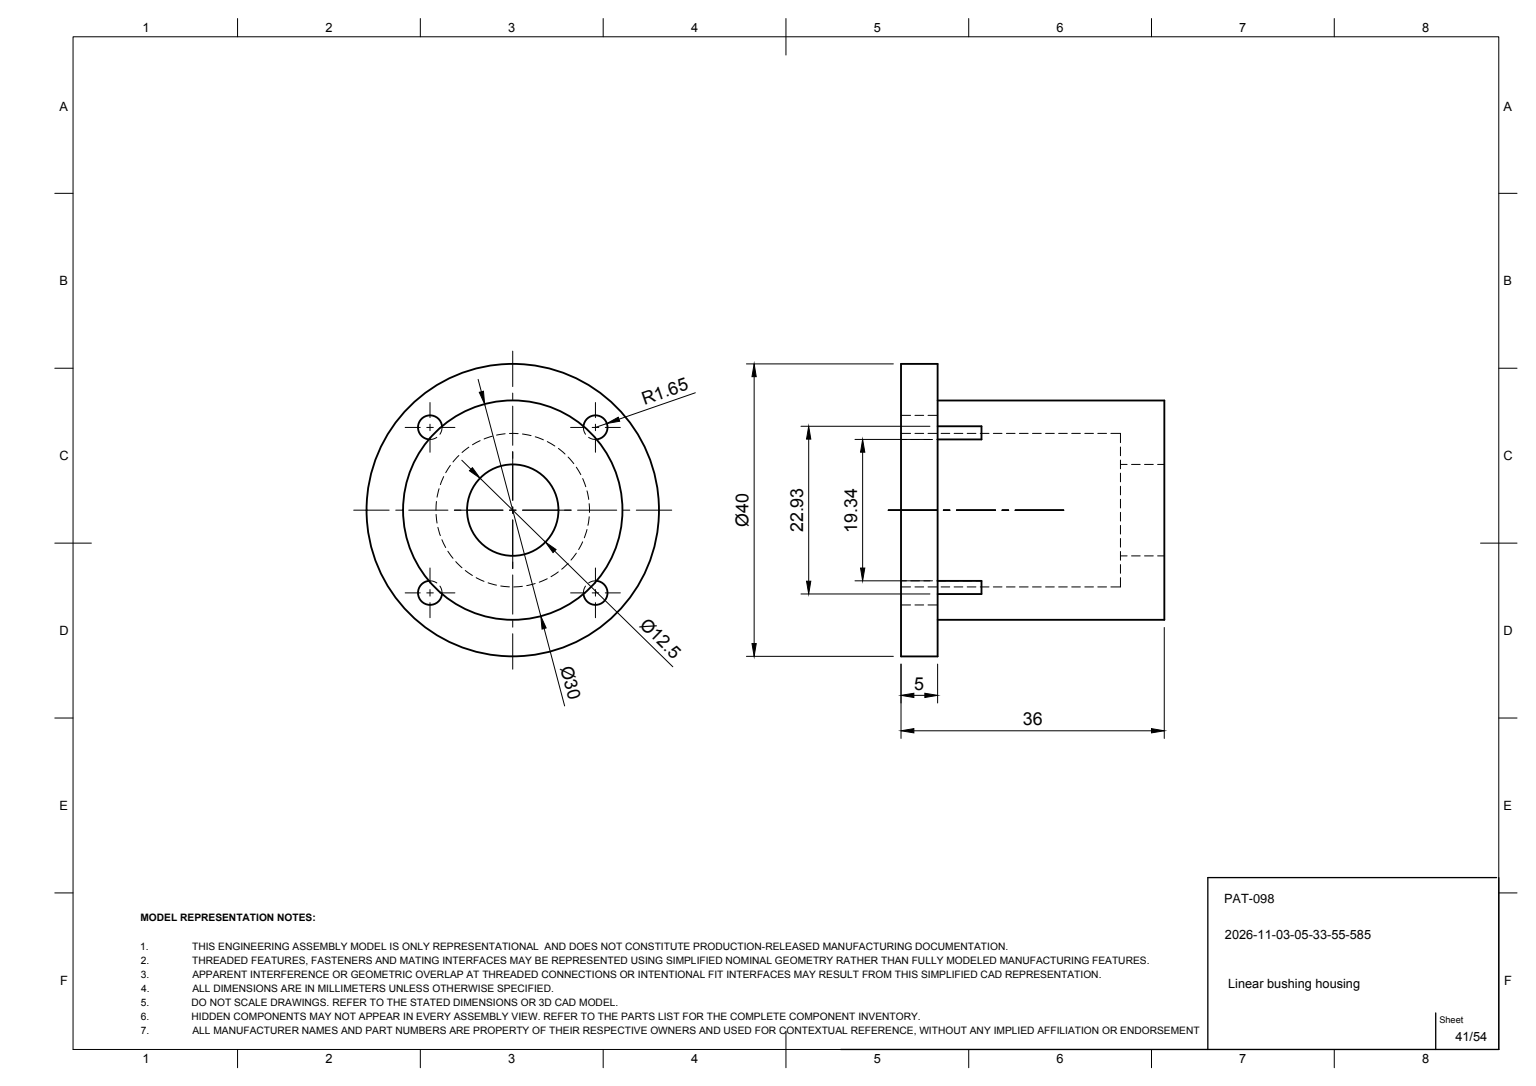
ISO-10303-21;
HEADER;
/* Generated by software containing ST-Developer
 * from STEP Tools, Inc. (www.steptools.com) 
 */

FILE_DESCRIPTION(
/* description */ ('Spring compression tester'),
/* implementation_level */ '2;1');

FILE_NAME(
/* name */ 'Linear bushing housing.step',
/* time_stamp */ '2026-10-28T03:24:11-07:00',
/* author */ (''),
/* organization */ (''),
/* preprocessor_version */ 'ST-DEVELOPER v20.2',
/* originating_system */ 'Autodesk Translation Framework v15.17.0.0',
/* authorisation */ '');

FILE_SCHEMA (('AUTOMOTIVE_DESIGN { 1 0 10303 214 3 1 1 }'));
ENDSEC;

DATA;
#10=MECHANICAL_DESIGN_GEOMETRIC_PRESENTATION_REPRESENTATION('',(#1159),#43521);
#1024=SHAPE_REPRESENTATION_RELATIONSHIP('SRR','None',#43839,#1084);
#1084=ADVANCED_BREP_SHAPE_REPRESENTATION('',(#1230),#43499);
#1159=STYLED_ITEM('',(#44181),#1230);
#1230=MANIFOLD_SOLID_BREP('Body1',#18600);
#1513=FACE_BOUND('',#4170,.T.);
#1514=FACE_BOUND('',#4172,.T.);
#1515=FACE_BOUND('',#4176,.T.);
#1516=FACE_BOUND('',#4177,.T.);
#1517=FACE_BOUND('',#4178,.T.);
#1518=FACE_BOUND('',#4179,.T.);
#1519=FACE_BOUND('',#4180,.T.);
#1520=FACE_BOUND('',#4182,.T.);
#2030=PLANE('',#20489);
#2031=PLANE('',#20496);
#2032=PLANE('',#20503);
#2033=PLANE('',#20510);
#2034=PLANE('',#20527);
#2035=PLANE('',#20529);
#2036=PLANE('',#20535);
#2037=PLANE('',#20536);
#2846=FACE_OUTER_BOUND('',#4159,.T.);
#2847=FACE_OUTER_BOUND('',#4160,.T.);
#2848=FACE_OUTER_BOUND('',#4161,.T.);
#2849=FACE_OUTER_BOUND('',#4162,.T.);
#2850=FACE_OUTER_BOUND('',#4163,.T.);
#2851=FACE_OUTER_BOUND('',#4164,.T.);
#2852=FACE_OUTER_BOUND('',#4165,.T.);
#2853=FACE_OUTER_BOUND('',#4166,.T.);
#2854=FACE_OUTER_BOUND('',#4167,.T.);
#2855=FACE_OUTER_BOUND('',#4168,.T.);
#2856=FACE_OUTER_BOUND('',#4169,.T.);
#2857=FACE_OUTER_BOUND('',#4171,.T.);
#2858=FACE_OUTER_BOUND('',#4173,.T.);
#2859=FACE_OUTER_BOUND('',#4174,.T.);
#2860=FACE_OUTER_BOUND('',#4175,.T.);
#2861=FACE_OUTER_BOUND('',#4181,.T.);
#4159=EDGE_LOOP('',(#15261,#15262));
#4160=EDGE_LOOP('',(#15263,#15264,#15265,#15266,#15267,#15268,#15269,#15270));
#4161=EDGE_LOOP('',(#15271,#15272));
#4162=EDGE_LOOP('',(#15273,#15274,#15275,#15276,#15277,#15278,#15279,#15280));
#4163=EDGE_LOOP('',(#15281,#15282,#15283));
#4164=EDGE_LOOP('',(#15284,#15285,#15286,#15287,#15288,#15289,#15290,#15291));
#4165=EDGE_LOOP('',(#15292,#15293,#15294));
#4166=EDGE_LOOP('',(#15295,#15296,#15297,#15298,#15299,#15300,#15301,#15302));
#4167=EDGE_LOOP('',(#15303,#15304,#15305,#15306,#15307,#15308,#15309,#15310,
#15311,#15312,#15313,#15314,#15315,#15316,#15317,#15318,#15319,#15320,#15321,
#15322));
#4168=EDGE_LOOP('',(#15323,#15324,#15325,#15326));
#4169=EDGE_LOOP('',(#15327));
#4170=EDGE_LOOP('',(#15328));
#4171=EDGE_LOOP('',(#15329));
#4172=EDGE_LOOP('',(#15330,#15331,#15332,#15333,#15334,#15335,#15336,#15337,
#15338,#15339,#15340));
#4173=EDGE_LOOP('',(#15341,#15342,#15343,#15344));
#4174=EDGE_LOOP('',(#15345,#15346,#15347,#15348));
#4175=EDGE_LOOP('',(#15349));
#4176=EDGE_LOOP('',(#15350));
#4177=EDGE_LOOP('',(#15351));
#4178=EDGE_LOOP('',(#15352));
#4179=EDGE_LOOP('',(#15353));
#4180=EDGE_LOOP('',(#15354));
#4181=EDGE_LOOP('',(#15355));
#4182=EDGE_LOOP('',(#15356));
#5623=LINE('',#30371,#7055);
#5624=LINE('',#30375,#7056);
#5625=LINE('',#30379,#7057);
#5626=LINE('',#30387,#7058);
#5627=LINE('',#30391,#7059);
#5628=LINE('',#30395,#7060);
#5629=LINE('',#30405,#7061);
#5630=LINE('',#30408,#7062);
#5631=LINE('',#30410,#7063);
#5632=LINE('',#30421,#7064);
#5633=LINE('',#30424,#7065);
#5634=LINE('',#30426,#7066);
#5635=LINE('',#30432,#7067);
#5636=LINE('',#30442,#7068);
#5637=LINE('',#30453,#7069);
#5638=LINE('',#30456,#7070);
#7055=VECTOR('',#24631,1.);
#7056=VECTOR('',#24634,0.165);
#7057=VECTOR('',#24639,1.);
#7058=VECTOR('',#24648,1.);
#7059=VECTOR('',#24651,0.165);
#7060=VECTOR('',#24656,1.);
#7061=VECTOR('',#24667,1.);
#7062=VECTOR('',#24670,1.);
#7063=VECTOR('',#24671,0.165);
#7064=VECTOR('',#24684,1.);
#7065=VECTOR('',#24687,1.);
#7066=VECTOR('',#24688,0.165);
#7067=VECTOR('',#24695,1.5);
#7068=VECTOR('',#24710,1.05);
#7069=VECTOR('',#24725,2.);
#7070=VECTOR('',#24728,0.625);
#7941=CIRCLE('',#20490,1.5);
#7942=CIRCLE('',#20491,0.165);
#7943=CIRCLE('',#20493,0.165);
#7944=CIRCLE('',#20494,0.165);
#7945=CIRCLE('',#20495,0.165);
#7946=CIRCLE('',#20497,1.5);
#7947=CIRCLE('',#20498,0.165);
#7948=CIRCLE('',#20500,0.165);
#7949=CIRCLE('',#20501,0.165);
#7950=CIRCLE('',#20502,0.165);
#7951=CIRCLE('',#20504,1.5);
#7952=CIRCLE('',#20505,0.165);
#7953=CIRCLE('',#20506,0.165);
#7954=CIRCLE('',#20508,0.165);
#7955=CIRCLE('',#20509,0.165);
#7956=CIRCLE('',#20511,1.5);
#7957=CIRCLE('',#20512,0.165);
#7958=CIRCLE('',#20513,0.165);
#7959=CIRCLE('',#20515,0.165);
#7960=CIRCLE('',#20516,0.165);
#7961=CIRCLE('',#20518,1.5);
#7962=CIRCLE('',#20519,1.5);
#7963=CIRCLE('',#20520,1.5);
#7964=CIRCLE('',#20521,1.5);
#7965=CIRCLE('',#20522,1.5);
#7966=CIRCLE('',#20523,1.5);
#7967=CIRCLE('',#20525,1.05);
#7968=CIRCLE('',#20526,1.05);
#7969=CIRCLE('',#20528,0.625);
#7970=CIRCLE('',#20530,2.);
#7971=CIRCLE('',#20532,2.);
#7972=CIRCLE('',#20534,0.625);
#9162=VERTEX_POINT('',#30365);
#9163=VERTEX_POINT('',#30366);
#9164=VERTEX_POINT('',#30370);
#9165=VERTEX_POINT('',#30372);
#9166=VERTEX_POINT('',#30374);
#9167=VERTEX_POINT('',#30377);
#9168=VERTEX_POINT('',#30381);
#9169=VERTEX_POINT('',#30382);
#9170=VERTEX_POINT('',#30386);
#9171=VERTEX_POINT('',#30388);
#9172=VERTEX_POINT('',#30390);
#9173=VERTEX_POINT('',#30393);
#9174=VERTEX_POINT('',#30397);
#9175=VERTEX_POINT('',#30398);
#9176=VERTEX_POINT('',#30400);
#9177=VERTEX_POINT('',#30404);
#9178=VERTEX_POINT('',#30406);
#9179=VERTEX_POINT('',#30409);
#9180=VERTEX_POINT('',#30413);
#9181=VERTEX_POINT('',#30414);
#9182=VERTEX_POINT('',#30416);
#9183=VERTEX_POINT('',#30420);
#9184=VERTEX_POINT('',#30422);
#9185=VERTEX_POINT('',#30425);
#9186=VERTEX_POINT('',#30429);
#9187=VERTEX_POINT('',#30431);
#9188=VERTEX_POINT('',#30439);
#9189=VERTEX_POINT('',#30441);
#9190=VERTEX_POINT('',#30445);
#9191=VERTEX_POINT('',#30448);
#9192=VERTEX_POINT('',#30451);
#9193=VERTEX_POINT('',#30455);
#11295=EDGE_CURVE('',#9162,#9163,#7941,.T.);
#11296=EDGE_CURVE('',#9162,#9163,#7942,.T.);
#11297=EDGE_CURVE('',#9164,#9162,#5623,.T.);
#11298=EDGE_CURVE('',#9165,#9164,#7943,.T.);
#11299=EDGE_CURVE('',#9165,#9166,#5624,.T.);
#11300=EDGE_CURVE('',#9166,#9166,#7944,.T.);
#11301=EDGE_CURVE('',#9167,#9165,#7945,.T.);
#11302=EDGE_CURVE('',#9163,#9167,#5625,.T.);
#11303=EDGE_CURVE('',#9168,#9169,#7946,.T.);
#11304=EDGE_CURVE('',#9168,#9169,#7947,.T.);
#11305=EDGE_CURVE('',#9170,#9168,#5626,.T.);
#11306=EDGE_CURVE('',#9171,#9170,#7948,.T.);
#11307=EDGE_CURVE('',#9171,#9172,#5627,.T.);
#11308=EDGE_CURVE('',#9172,#9172,#7949,.T.);
#11309=EDGE_CURVE('',#9173,#9171,#7950,.T.);
#11310=EDGE_CURVE('',#9169,#9173,#5628,.T.);
#11311=EDGE_CURVE('',#9174,#9175,#7951,.T.);
#11312=EDGE_CURVE('',#9174,#9176,#7952,.T.);
#11313=EDGE_CURVE('',#9176,#9175,#7953,.T.);
#11314=EDGE_CURVE('',#9177,#9174,#5629,.T.);
#11315=EDGE_CURVE('',#9178,#9177,#7954,.T.);
#11316=EDGE_CURVE('',#9175,#9178,#5630,.T.);
#11317=EDGE_CURVE('',#9176,#9179,#5631,.T.);
#11318=EDGE_CURVE('',#9179,#9179,#7955,.T.);
#11319=EDGE_CURVE('',#9180,#9181,#7956,.T.);
#11320=EDGE_CURVE('',#9180,#9182,#7957,.T.);
#11321=EDGE_CURVE('',#9182,#9181,#7958,.T.);
#11322=EDGE_CURVE('',#9183,#9180,#5632,.T.);
#11323=EDGE_CURVE('',#9184,#9183,#7959,.T.);
#11324=EDGE_CURVE('',#9181,#9184,#5633,.T.);
#11325=EDGE_CURVE('',#9182,#9185,#5634,.T.);
#11326=EDGE_CURVE('',#9185,#9185,#7960,.T.);
#11327=EDGE_CURVE('',#9167,#9186,#7961,.T.);
#11328=EDGE_CURVE('',#9186,#9187,#5635,.T.);
#11329=EDGE_CURVE('',#9187,#9187,#7962,.T.);
#11330=EDGE_CURVE('',#9186,#9170,#7963,.T.);
#11331=EDGE_CURVE('',#9173,#9177,#7964,.T.);
#11332=EDGE_CURVE('',#9178,#9183,#7965,.T.);
#11333=EDGE_CURVE('',#9184,#9164,#7966,.T.);
#11334=EDGE_CURVE('',#9188,#9188,#7967,.T.);
#11335=EDGE_CURVE('',#9188,#9189,#5636,.T.);
#11336=EDGE_CURVE('',#9189,#9189,#7968,.T.);
#11337=EDGE_CURVE('',#9190,#9190,#7969,.T.);
#11338=EDGE_CURVE('',#9191,#9191,#7970,.T.);
#11339=EDGE_CURVE('',#9192,#9192,#7971,.T.);
#11340=EDGE_CURVE('',#9192,#9191,#5637,.T.);
#11341=EDGE_CURVE('',#9190,#9193,#5638,.T.);
#11342=EDGE_CURVE('',#9193,#9193,#7972,.T.);
#15261=ORIENTED_EDGE('',*,*,#11295,.F.);
#15262=ORIENTED_EDGE('',*,*,#11296,.T.);
#15263=ORIENTED_EDGE('',*,*,#11297,.F.);
#15264=ORIENTED_EDGE('',*,*,#11298,.F.);
#15265=ORIENTED_EDGE('',*,*,#11299,.T.);
#15266=ORIENTED_EDGE('',*,*,#11300,.F.);
#15267=ORIENTED_EDGE('',*,*,#11299,.F.);
#15268=ORIENTED_EDGE('',*,*,#11301,.F.);
#15269=ORIENTED_EDGE('',*,*,#11302,.F.);
#15270=ORIENTED_EDGE('',*,*,#11296,.F.);
#15271=ORIENTED_EDGE('',*,*,#11303,.F.);
#15272=ORIENTED_EDGE('',*,*,#11304,.T.);
#15273=ORIENTED_EDGE('',*,*,#11305,.F.);
#15274=ORIENTED_EDGE('',*,*,#11306,.F.);
#15275=ORIENTED_EDGE('',*,*,#11307,.T.);
#15276=ORIENTED_EDGE('',*,*,#11308,.F.);
#15277=ORIENTED_EDGE('',*,*,#11307,.F.);
#15278=ORIENTED_EDGE('',*,*,#11309,.F.);
#15279=ORIENTED_EDGE('',*,*,#11310,.F.);
#15280=ORIENTED_EDGE('',*,*,#11304,.F.);
#15281=ORIENTED_EDGE('',*,*,#11311,.F.);
#15282=ORIENTED_EDGE('',*,*,#11312,.T.);
#15283=ORIENTED_EDGE('',*,*,#11313,.T.);
#15284=ORIENTED_EDGE('',*,*,#11314,.F.);
#15285=ORIENTED_EDGE('',*,*,#11315,.F.);
#15286=ORIENTED_EDGE('',*,*,#11316,.F.);
#15287=ORIENTED_EDGE('',*,*,#11313,.F.);
#15288=ORIENTED_EDGE('',*,*,#11317,.T.);
#15289=ORIENTED_EDGE('',*,*,#11318,.F.);
#15290=ORIENTED_EDGE('',*,*,#11317,.F.);
#15291=ORIENTED_EDGE('',*,*,#11312,.F.);
#15292=ORIENTED_EDGE('',*,*,#11319,.F.);
#15293=ORIENTED_EDGE('',*,*,#11320,.T.);
#15294=ORIENTED_EDGE('',*,*,#11321,.T.);
#15295=ORIENTED_EDGE('',*,*,#11322,.F.);
#15296=ORIENTED_EDGE('',*,*,#11323,.F.);
#15297=ORIENTED_EDGE('',*,*,#11324,.F.);
#15298=ORIENTED_EDGE('',*,*,#11321,.F.);
#15299=ORIENTED_EDGE('',*,*,#11325,.T.);
#15300=ORIENTED_EDGE('',*,*,#11326,.F.);
#15301=ORIENTED_EDGE('',*,*,#11325,.F.);
#15302=ORIENTED_EDGE('',*,*,#11320,.F.);
#15303=ORIENTED_EDGE('',*,*,#11297,.T.);
#15304=ORIENTED_EDGE('',*,*,#11295,.T.);
#15305=ORIENTED_EDGE('',*,*,#11302,.T.);
#15306=ORIENTED_EDGE('',*,*,#11327,.T.);
#15307=ORIENTED_EDGE('',*,*,#11328,.T.);
#15308=ORIENTED_EDGE('',*,*,#11329,.T.);
#15309=ORIENTED_EDGE('',*,*,#11328,.F.);
#15310=ORIENTED_EDGE('',*,*,#11330,.T.);
#15311=ORIENTED_EDGE('',*,*,#11305,.T.);
#15312=ORIENTED_EDGE('',*,*,#11303,.T.);
#15313=ORIENTED_EDGE('',*,*,#11310,.T.);
#15314=ORIENTED_EDGE('',*,*,#11331,.T.);
#15315=ORIENTED_EDGE('',*,*,#11314,.T.);
#15316=ORIENTED_EDGE('',*,*,#11311,.T.);
#15317=ORIENTED_EDGE('',*,*,#11316,.T.);
#15318=ORIENTED_EDGE('',*,*,#11332,.T.);
#15319=ORIENTED_EDGE('',*,*,#11322,.T.);
#15320=ORIENTED_EDGE('',*,*,#11319,.T.);
#15321=ORIENTED_EDGE('',*,*,#11324,.T.);
#15322=ORIENTED_EDGE('',*,*,#11333,.T.);
#15323=ORIENTED_EDGE('',*,*,#11334,.F.);
#15324=ORIENTED_EDGE('',*,*,#11335,.T.);
#15325=ORIENTED_EDGE('',*,*,#11336,.F.);
#15326=ORIENTED_EDGE('',*,*,#11335,.F.);
#15327=ORIENTED_EDGE('',*,*,#11334,.T.);
#15328=ORIENTED_EDGE('',*,*,#11337,.F.);
#15329=ORIENTED_EDGE('',*,*,#11338,.F.);
#15330=ORIENTED_EDGE('',*,*,#11301,.T.);
#15331=ORIENTED_EDGE('',*,*,#11298,.T.);
#15332=ORIENTED_EDGE('',*,*,#11333,.F.);
#15333=ORIENTED_EDGE('',*,*,#11323,.T.);
#15334=ORIENTED_EDGE('',*,*,#11332,.F.);
#15335=ORIENTED_EDGE('',*,*,#11315,.T.);
#15336=ORIENTED_EDGE('',*,*,#11331,.F.);
#15337=ORIENTED_EDGE('',*,*,#11309,.T.);
#15338=ORIENTED_EDGE('',*,*,#11306,.T.);
#15339=ORIENTED_EDGE('',*,*,#11330,.F.);
#15340=ORIENTED_EDGE('',*,*,#11327,.F.);
#15341=ORIENTED_EDGE('',*,*,#11339,.F.);
#15342=ORIENTED_EDGE('',*,*,#11340,.T.);
#15343=ORIENTED_EDGE('',*,*,#11338,.T.);
#15344=ORIENTED_EDGE('',*,*,#11340,.F.);
#15345=ORIENTED_EDGE('',*,*,#11337,.T.);
#15346=ORIENTED_EDGE('',*,*,#11341,.T.);
#15347=ORIENTED_EDGE('',*,*,#11342,.T.);
#15348=ORIENTED_EDGE('',*,*,#11341,.F.);
#15349=ORIENTED_EDGE('',*,*,#11339,.T.);
#15350=ORIENTED_EDGE('',*,*,#11336,.T.);
#15351=ORIENTED_EDGE('',*,*,#11326,.T.);
#15352=ORIENTED_EDGE('',*,*,#11318,.T.);
#15353=ORIENTED_EDGE('',*,*,#11308,.T.);
#15354=ORIENTED_EDGE('',*,*,#11300,.T.);
#15355=ORIENTED_EDGE('',*,*,#11329,.F.);
#15356=ORIENTED_EDGE('',*,*,#11342,.F.);
#17280=CYLINDRICAL_SURFACE('',#20492,0.165);
#17281=CYLINDRICAL_SURFACE('',#20499,0.165);
#17282=CYLINDRICAL_SURFACE('',#20507,0.165);
#17283=CYLINDRICAL_SURFACE('',#20514,0.165);
#17284=CYLINDRICAL_SURFACE('',#20517,1.5);
#17285=CYLINDRICAL_SURFACE('',#20524,1.05);
#17286=CYLINDRICAL_SURFACE('',#20531,2.);
#17287=CYLINDRICAL_SURFACE('',#20533,0.625);
#18170=ADVANCED_FACE('',(#2846),#2030,.T.);
#18171=ADVANCED_FACE('',(#2847),#17280,.F.);
#18172=ADVANCED_FACE('',(#2848),#2031,.T.);
#18173=ADVANCED_FACE('',(#2849),#17281,.F.);
#18174=ADVANCED_FACE('',(#2850),#2032,.T.);
#18175=ADVANCED_FACE('',(#2851),#17282,.F.);
#18176=ADVANCED_FACE('',(#2852),#2033,.T.);
#18177=ADVANCED_FACE('',(#2853),#17283,.F.);
#18178=ADVANCED_FACE('',(#2854),#17284,.T.);
#18179=ADVANCED_FACE('',(#2855),#17285,.F.);
#18180=ADVANCED_FACE('',(#2856,#1513),#2034,.T.);
#18181=ADVANCED_FACE('',(#2857,#1514),#2035,.F.);
#18182=ADVANCED_FACE('',(#2858),#17286,.T.);
#18183=ADVANCED_FACE('',(#2859),#17287,.F.);
#18184=ADVANCED_FACE('',(#2860,#1515,#1516,#1517,#1518,#1519),#2036,.T.);
#18185=ADVANCED_FACE('',(#2861,#1520),#2037,.F.);
#18600=CLOSED_SHELL('',(#18170,#18171,#18172,#18173,#18174,#18175,#18176,
#18177,#18178,#18179,#18180,#18181,#18182,#18183,#18184,#18185));
#20488=AXIS2_PLACEMENT_3D('',#30363,#24621,#24622);
#20489=AXIS2_PLACEMENT_3D('',#30364,#24623,#24624);
#20490=AXIS2_PLACEMENT_3D('',#30367,#24625,#24626);
#20491=AXIS2_PLACEMENT_3D('',#30368,#24627,#24628);
#20492=AXIS2_PLACEMENT_3D('',#30369,#24629,#24630);
#20493=AXIS2_PLACEMENT_3D('',#30373,#24632,#24633);
#20494=AXIS2_PLACEMENT_3D('',#30376,#24635,#24636);
#20495=AXIS2_PLACEMENT_3D('',#30378,#24637,#24638);
#20496=AXIS2_PLACEMENT_3D('',#30380,#24640,#24641);
#20497=AXIS2_PLACEMENT_3D('',#30383,#24642,#24643);
#20498=AXIS2_PLACEMENT_3D('',#30384,#24644,#24645);
#20499=AXIS2_PLACEMENT_3D('',#30385,#24646,#24647);
#20500=AXIS2_PLACEMENT_3D('',#30389,#24649,#24650);
#20501=AXIS2_PLACEMENT_3D('',#30392,#24652,#24653);
#20502=AXIS2_PLACEMENT_3D('',#30394,#24654,#24655);
#20503=AXIS2_PLACEMENT_3D('',#30396,#24657,#24658);
#20504=AXIS2_PLACEMENT_3D('',#30399,#24659,#24660);
#20505=AXIS2_PLACEMENT_3D('',#30401,#24661,#24662);
#20506=AXIS2_PLACEMENT_3D('',#30402,#24663,#24664);
#20507=AXIS2_PLACEMENT_3D('',#30403,#24665,#24666);
#20508=AXIS2_PLACEMENT_3D('',#30407,#24668,#24669);
#20509=AXIS2_PLACEMENT_3D('',#30411,#24672,#24673);
#20510=AXIS2_PLACEMENT_3D('',#30412,#24674,#24675);
#20511=AXIS2_PLACEMENT_3D('',#30415,#24676,#24677);
#20512=AXIS2_PLACEMENT_3D('',#30417,#24678,#24679);
#20513=AXIS2_PLACEMENT_3D('',#30418,#24680,#24681);
#20514=AXIS2_PLACEMENT_3D('',#30419,#24682,#24683);
#20515=AXIS2_PLACEMENT_3D('',#30423,#24685,#24686);
#20516=AXIS2_PLACEMENT_3D('',#30427,#24689,#24690);
#20517=AXIS2_PLACEMENT_3D('',#30428,#24691,#24692);
#20518=AXIS2_PLACEMENT_3D('',#30430,#24693,#24694);
#20519=AXIS2_PLACEMENT_3D('',#30433,#24696,#24697);
#20520=AXIS2_PLACEMENT_3D('',#30434,#24698,#24699);
#20521=AXIS2_PLACEMENT_3D('',#30435,#24700,#24701);
#20522=AXIS2_PLACEMENT_3D('',#30436,#24702,#24703);
#20523=AXIS2_PLACEMENT_3D('',#30437,#24704,#24705);
#20524=AXIS2_PLACEMENT_3D('',#30438,#24706,#24707);
#20525=AXIS2_PLACEMENT_3D('',#30440,#24708,#24709);
#20526=AXIS2_PLACEMENT_3D('',#30443,#24711,#24712);
#20527=AXIS2_PLACEMENT_3D('',#30444,#24713,#24714);
#20528=AXIS2_PLACEMENT_3D('',#30446,#24715,#24716);
#20529=AXIS2_PLACEMENT_3D('',#30447,#24717,#24718);
#20530=AXIS2_PLACEMENT_3D('',#30449,#24719,#24720);
#20531=AXIS2_PLACEMENT_3D('',#30450,#24721,#24722);
#20532=AXIS2_PLACEMENT_3D('',#30452,#24723,#24724);
#20533=AXIS2_PLACEMENT_3D('',#30454,#24726,#24727);
#20534=AXIS2_PLACEMENT_3D('',#30457,#24729,#24730);
#20535=AXIS2_PLACEMENT_3D('',#30458,#24731,#24732);
#20536=AXIS2_PLACEMENT_3D('',#30459,#24733,#24734);
#24621=DIRECTION('axis',(0.,0.,1.));
#24622=DIRECTION('refdir',(1.,0.,0.));
#24623=DIRECTION('center_axis',(0.,0.,1.));
#24624=DIRECTION('ref_axis',(1.,0.,0.));
#24625=DIRECTION('center_axis',(0.,0.,-1.));
#24626=DIRECTION('ref_axis',(1.,0.,0.));
#24627=DIRECTION('center_axis',(0.,0.,1.));
#24628=DIRECTION('ref_axis',(1.,0.,0.));
#24629=DIRECTION('center_axis',(0.,0.,1.));
#24630=DIRECTION('ref_axis',(1.,0.,0.));
#24631=DIRECTION('',(0.,0.,-1.));
#24632=DIRECTION('center_axis',(0.,0.,1.));
#24633=DIRECTION('ref_axis',(1.,0.,0.));
#24634=DIRECTION('',(0.,0.,1.));
#24635=DIRECTION('center_axis',(0.,0.,-1.));
#24636=DIRECTION('ref_axis',(1.,0.,0.));
#24637=DIRECTION('center_axis',(0.,0.,1.));
#24638=DIRECTION('ref_axis',(1.,0.,0.));
#24639=DIRECTION('',(0.,0.,1.));
#24640=DIRECTION('center_axis',(0.,0.,1.));
#24641=DIRECTION('ref_axis',(1.,0.,0.));
#24642=DIRECTION('center_axis',(0.,0.,-1.));
#24643=DIRECTION('ref_axis',(1.,0.,0.));
#24644=DIRECTION('center_axis',(0.,0.,1.));
#24645=DIRECTION('ref_axis',(1.,0.,0.));
#24646=DIRECTION('center_axis',(0.,0.,1.));
#24647=DIRECTION('ref_axis',(1.,0.,0.));
#24648=DIRECTION('',(0.,0.,-1.));
#24649=DIRECTION('center_axis',(0.,0.,1.));
#24650=DIRECTION('ref_axis',(1.,0.,0.));
#24651=DIRECTION('',(0.,0.,1.));
#24652=DIRECTION('center_axis',(0.,0.,-1.));
#24653=DIRECTION('ref_axis',(1.,0.,0.));
#24654=DIRECTION('center_axis',(0.,0.,1.));
#24655=DIRECTION('ref_axis',(1.,0.,0.));
#24656=DIRECTION('',(0.,0.,1.));
#24657=DIRECTION('center_axis',(0.,0.,1.));
#24658=DIRECTION('ref_axis',(1.,0.,0.));
#24659=DIRECTION('center_axis',(0.,0.,-1.));
#24660=DIRECTION('ref_axis',(1.,0.,0.));
#24661=DIRECTION('center_axis',(0.,0.,1.));
#24662=DIRECTION('ref_axis',(1.,0.,0.));
#24663=DIRECTION('center_axis',(0.,0.,1.));
#24664=DIRECTION('ref_axis',(1.,0.,0.));
#24665=DIRECTION('center_axis',(0.,0.,1.));
#24666=DIRECTION('ref_axis',(1.,0.,0.));
#24667=DIRECTION('',(0.,0.,-1.));
#24668=DIRECTION('center_axis',(0.,0.,1.));
#24669=DIRECTION('ref_axis',(1.,0.,0.));
#24670=DIRECTION('',(0.,0.,1.));
#24671=DIRECTION('',(0.,0.,1.));
#24672=DIRECTION('center_axis',(0.,0.,-1.));
#24673=DIRECTION('ref_axis',(1.,0.,0.));
#24674=DIRECTION('center_axis',(0.,0.,1.));
#24675=DIRECTION('ref_axis',(1.,0.,0.));
#24676=DIRECTION('center_axis',(0.,0.,-1.));
#24677=DIRECTION('ref_axis',(1.,0.,0.));
#24678=DIRECTION('center_axis',(0.,0.,1.));
#24679=DIRECTION('ref_axis',(1.,0.,0.));
#24680=DIRECTION('center_axis',(0.,0.,1.));
#24681=DIRECTION('ref_axis',(1.,0.,0.));
#24682=DIRECTION('center_axis',(0.,0.,1.));
#24683=DIRECTION('ref_axis',(1.,0.,0.));
#24684=DIRECTION('',(0.,0.,-1.));
#24685=DIRECTION('center_axis',(0.,0.,1.));
#24686=DIRECTION('ref_axis',(1.,0.,0.));
#24687=DIRECTION('',(0.,0.,1.));
#24688=DIRECTION('',(0.,0.,1.));
#24689=DIRECTION('center_axis',(0.,0.,-1.));
#24690=DIRECTION('ref_axis',(1.,0.,0.));
#24691=DIRECTION('center_axis',(0.,0.,1.));
#24692=DIRECTION('ref_axis',(1.,0.,0.));
#24693=DIRECTION('center_axis',(0.,0.,-1.));
#24694=DIRECTION('ref_axis',(1.,0.,0.));
#24695=DIRECTION('',(0.,0.,-1.));
#24696=DIRECTION('center_axis',(0.,0.,1.));
#24697=DIRECTION('ref_axis',(1.,0.,0.));
#24698=DIRECTION('center_axis',(0.,0.,-1.));
#24699=DIRECTION('ref_axis',(1.,0.,0.));
#24700=DIRECTION('center_axis',(0.,0.,-1.));
#24701=DIRECTION('ref_axis',(1.,0.,0.));
#24702=DIRECTION('center_axis',(0.,0.,-1.));
#24703=DIRECTION('ref_axis',(1.,0.,0.));
#24704=DIRECTION('center_axis',(0.,0.,-1.));
#24705=DIRECTION('ref_axis',(1.,0.,0.));
#24706=DIRECTION('center_axis',(0.,0.,1.));
#24707=DIRECTION('ref_axis',(1.,0.,0.));
#24708=DIRECTION('center_axis',(0.,0.,1.));
#24709=DIRECTION('ref_axis',(1.,0.,0.));
#24710=DIRECTION('',(0.,0.,1.));
#24711=DIRECTION('center_axis',(0.,0.,-1.));
#24712=DIRECTION('ref_axis',(1.,0.,0.));
#24713=DIRECTION('center_axis',(0.,0.,1.));
#24714=DIRECTION('ref_axis',(1.,0.,0.));
#24715=DIRECTION('center_axis',(0.,0.,1.));
#24716=DIRECTION('ref_axis',(1.,0.,0.));
#24717=DIRECTION('center_axis',(0.,0.,1.));
#24718=DIRECTION('ref_axis',(1.,0.,0.));
#24719=DIRECTION('center_axis',(0.,0.,1.));
#24720=DIRECTION('ref_axis',(1.,0.,0.));
#24721=DIRECTION('center_axis',(0.,0.,1.));
#24722=DIRECTION('ref_axis',(1.,0.,0.));
#24723=DIRECTION('center_axis',(0.,0.,1.));
#24724=DIRECTION('ref_axis',(1.,0.,0.));
#24725=DIRECTION('',(0.,0.,-1.));
#24726=DIRECTION('center_axis',(0.,0.,1.));
#24727=DIRECTION('ref_axis',(1.,0.,0.));
#24728=DIRECTION('',(0.,0.,-1.));
#24729=DIRECTION('center_axis',(0.,0.,-1.));
#24730=DIRECTION('ref_axis',(1.,0.,0.));
#24731=DIRECTION('center_axis',(0.,0.,1.));
#24732=DIRECTION('ref_axis',(1.,0.,0.));
#24733=DIRECTION('center_axis',(0.,0.,1.));
#24734=DIRECTION('ref_axis',(1.,0.,0.));
#30363=CARTESIAN_POINT('',(0.,0.,0.));
#30364=CARTESIAN_POINT('Origin',(-7.13137084989848,-1.13137084989848,14.));
#30365=CARTESIAN_POINT('',(-6.96707794165985,-1.14662995545858,14.));
#30366=CARTESIAN_POINT('',(-7.14662995545858,-0.96707794165985,14.));
#30367=CARTESIAN_POINT('Origin',(-6.,0.,14.));
#30368=CARTESIAN_POINT('Origin',(-7.13137084989848,-1.13137084989848,14.));
#30369=CARTESIAN_POINT('Origin',(-7.13137084989848,-1.13137084989848,14.));
#30370=CARTESIAN_POINT('',(-6.96707794165985,-1.14662995545858,14.6));
#30371=CARTESIAN_POINT('',(-6.96707794165985,-1.14662995545858,14.));
#30372=CARTESIAN_POINT('',(-7.29637084989848,-1.13137084989848,14.6));
#30373=CARTESIAN_POINT('Origin',(-7.13137084989848,-1.13137084989848,14.6));
#30374=CARTESIAN_POINT('',(-7.29637084989848,-1.13137084989848,15.1));
#30375=CARTESIAN_POINT('',(-7.29637084989848,-1.13137084989848,14.));
#30376=CARTESIAN_POINT('Origin',(-7.13137084989848,-1.13137084989848,15.1));
#30377=CARTESIAN_POINT('',(-7.14662995545858,-0.967077941659851,14.6));
#30378=CARTESIAN_POINT('Origin',(-7.13137084989848,-1.13137084989848,14.6));
#30379=CARTESIAN_POINT('',(-7.14662995545858,-0.96707794165985,14.));
#30380=CARTESIAN_POINT('Origin',(-7.13137084989848,1.13137084989848,14.));
#30381=CARTESIAN_POINT('',(-7.14662995545858,0.96707794165985,14.));
#30382=CARTESIAN_POINT('',(-6.96707794165985,1.14662995545858,14.));
#30383=CARTESIAN_POINT('Origin',(-6.,0.,14.));
#30384=CARTESIAN_POINT('Origin',(-7.13137084989848,1.13137084989848,14.));
#30385=CARTESIAN_POINT('Origin',(-7.13137084989848,1.13137084989848,14.));
#30386=CARTESIAN_POINT('',(-7.14662995545858,0.967077941659851,14.6));
#30387=CARTESIAN_POINT('',(-7.14662995545858,0.96707794165985,14.));
#30388=CARTESIAN_POINT('',(-7.29637084989848,1.13137084989848,14.6));
#30389=CARTESIAN_POINT('Origin',(-7.13137084989848,1.13137084989848,14.6));
#30390=CARTESIAN_POINT('',(-7.29637084989848,1.13137084989848,15.1));
#30391=CARTESIAN_POINT('',(-7.29637084989848,1.13137084989848,14.));
#30392=CARTESIAN_POINT('Origin',(-7.13137084989848,1.13137084989848,15.1));
#30393=CARTESIAN_POINT('',(-6.96707794165985,1.14662995545858,14.6));
#30394=CARTESIAN_POINT('Origin',(-7.13137084989848,1.13137084989848,14.6));
#30395=CARTESIAN_POINT('',(-6.96707794165985,1.14662995545858,14.));
#30396=CARTESIAN_POINT('Origin',(-4.86862915010152,1.13137084989848,14.));
#30397=CARTESIAN_POINT('',(-5.03292205834015,1.14662995545858,14.));
#30398=CARTESIAN_POINT('',(-4.85337004454142,0.96707794165985,14.));
#30399=CARTESIAN_POINT('Origin',(-6.,0.,14.));
#30400=CARTESIAN_POINT('',(-5.03362915010152,1.13137084989848,14.));
#30401=CARTESIAN_POINT('Origin',(-4.86862915010152,1.13137084989848,14.));
#30402=CARTESIAN_POINT('Origin',(-4.86862915010152,1.13137084989848,14.));
#30403=CARTESIAN_POINT('Origin',(-4.86862915010152,1.13137084989848,14.));
#30404=CARTESIAN_POINT('',(-5.03292205834015,1.14662995545858,14.6));
#30405=CARTESIAN_POINT('',(-5.03292205834015,1.14662995545858,14.));
#30406=CARTESIAN_POINT('',(-4.85337004454142,0.967077941659849,14.6));
#30407=CARTESIAN_POINT('Origin',(-4.86862915010152,1.13137084989848,14.6));
#30408=CARTESIAN_POINT('',(-4.85337004454142,0.96707794165985,14.));
#30409=CARTESIAN_POINT('',(-5.03362915010152,1.13137084989848,15.1));
#30410=CARTESIAN_POINT('',(-5.03362915010152,1.13137084989848,14.));
#30411=CARTESIAN_POINT('Origin',(-4.86862915010152,1.13137084989848,15.1));
#30412=CARTESIAN_POINT('Origin',(-4.86862915010152,-1.13137084989848,14.));
#30413=CARTESIAN_POINT('',(-4.85337004454142,-0.96707794165985,14.));
#30414=CARTESIAN_POINT('',(-5.03292205834015,-1.14662995545858,14.));
#30415=CARTESIAN_POINT('Origin',(-6.,0.,14.));
#30416=CARTESIAN_POINT('',(-5.03362915010152,-1.13137084989848,14.));
#30417=CARTESIAN_POINT('Origin',(-4.86862915010152,-1.13137084989848,14.));
#30418=CARTESIAN_POINT('Origin',(-4.86862915010152,-1.13137084989848,14.));
#30419=CARTESIAN_POINT('Origin',(-4.86862915010152,-1.13137084989848,14.));
#30420=CARTESIAN_POINT('',(-4.85337004454142,-0.967077941659849,14.6));
#30421=CARTESIAN_POINT('',(-4.85337004454142,-0.96707794165985,14.));
#30422=CARTESIAN_POINT('',(-5.03292205834015,-1.14662995545858,14.6));
#30423=CARTESIAN_POINT('Origin',(-4.86862915010152,-1.13137084989848,14.6));
#30424=CARTESIAN_POINT('',(-5.03292205834015,-1.14662995545858,14.));
#30425=CARTESIAN_POINT('',(-5.03362915010152,-1.13137084989848,15.1));
#30426=CARTESIAN_POINT('',(-5.03362915010152,-1.13137084989848,14.));
#30427=CARTESIAN_POINT('Origin',(-4.86862915010152,-1.13137084989848,15.1));
#30428=CARTESIAN_POINT('Origin',(-6.,0.,11.5));
#30429=CARTESIAN_POINT('',(-7.5,-1.83697019872103E-16,14.6));
#30430=CARTESIAN_POINT('Origin',(-6.,0.,14.6));
#30431=CARTESIAN_POINT('',(-7.5,-1.83697019872103E-16,11.5));
#30432=CARTESIAN_POINT('',(-7.5,-1.83697019872103E-16,11.5));
#30433=CARTESIAN_POINT('Origin',(-6.,0.,11.5));
#30434=CARTESIAN_POINT('Origin',(-6.,0.,14.6));
#30435=CARTESIAN_POINT('Origin',(-6.,0.,14.6));
#30436=CARTESIAN_POINT('Origin',(-6.,0.,14.6));
#30437=CARTESIAN_POINT('Origin',(-6.,0.,14.6));
#30438=CARTESIAN_POINT('Origin',(-6.,0.,12.1));
#30439=CARTESIAN_POINT('',(-7.05,-1.28587913910472E-16,12.1));
#30440=CARTESIAN_POINT('Origin',(-6.,0.,12.1));
#30441=CARTESIAN_POINT('',(-7.05,1.28587913910472E-16,15.1));
#30442=CARTESIAN_POINT('',(-7.05,-1.28587913910472E-16,12.1));
#30443=CARTESIAN_POINT('Origin',(-6.,0.,15.1));
#30444=CARTESIAN_POINT('Origin',(-6.,0.,12.1));
#30445=CARTESIAN_POINT('',(-6.625,-7.65404249467096E-17,12.1));
#30446=CARTESIAN_POINT('Origin',(-6.,0.,12.1));
#30447=CARTESIAN_POINT('Origin',(-6.,0.,14.6));
#30448=CARTESIAN_POINT('',(-8.,-2.44929359829471E-16,14.6));
#30449=CARTESIAN_POINT('Origin',(-6.,0.,14.6));
#30450=CARTESIAN_POINT('Origin',(-6.,0.,14.6));
#30451=CARTESIAN_POINT('',(-8.,-2.44929359829471E-16,15.1));
#30452=CARTESIAN_POINT('Origin',(-6.,0.,15.1));
#30453=CARTESIAN_POINT('',(-8.,-2.44929359829471E-16,14.6));
#30454=CARTESIAN_POINT('Origin',(-6.,0.,11.5));
#30455=CARTESIAN_POINT('',(-6.625,-7.65404249467096E-17,11.5));
#30456=CARTESIAN_POINT('',(-6.625,-7.65404249467096E-17,11.5));
#30457=CARTESIAN_POINT('Origin',(-6.,0.,11.5));
#30458=CARTESIAN_POINT('Origin',(-6.,0.,15.1));
#30459=CARTESIAN_POINT('Origin',(-6.,0.,11.5));
#43431=UNCERTAINTY_MEASURE_WITH_UNIT(LENGTH_MEASURE(0.001),#43522,
'DISTANCE_ACCURACY_VALUE',
'Maximum model space distance between geometric entities at asserted c
onnectivities');
#43453=UNCERTAINTY_MEASURE_WITH_UNIT(LENGTH_MEASURE(0.001),#43522,
'DISTANCE_ACCURACY_VALUE',
'Maximum model space distance between geometric entities at asserted c
onnectivities');
#43499=(
GEOMETRIC_REPRESENTATION_CONTEXT(3)
GLOBAL_UNCERTAINTY_ASSIGNED_CONTEXT((#43431))
GLOBAL_UNIT_ASSIGNED_CONTEXT((#43522,#43524,#43525))
REPRESENTATION_CONTEXT('','3D')
);
#43521=(
GEOMETRIC_REPRESENTATION_CONTEXT(3)
GLOBAL_UNCERTAINTY_ASSIGNED_CONTEXT((#43453))
GLOBAL_UNIT_ASSIGNED_CONTEXT((#43522,#43524,#43525))
REPRESENTATION_CONTEXT('','3D')
);
#43522=(
LENGTH_UNIT()
NAMED_UNIT(*)
SI_UNIT(.CENTI.,.METRE.)
);
#43524=(
NAMED_UNIT(*)
PLANE_ANGLE_UNIT()
SI_UNIT($,.RADIAN.)
);
#43525=(
NAMED_UNIT(*)
SI_UNIT($,.STERADIAN.)
SOLID_ANGLE_UNIT()
);
#43571=SHAPE_DEFINITION_REPRESENTATION(#43648,#43839);
#43648=PRODUCT_DEFINITION_SHAPE('',$,#43907);
#43839=SHAPE_REPRESENTATION('',(#20488),#43499);
#43861=PRODUCT_DEFINITION_CONTEXT('part definition',#44064,'design');
#43907=PRODUCT_DEFINITION('Linear bushing housing',
'Linear bushing housing',#43974,#43861);
#43974=PRODUCT_DEFINITION_FORMATION('',$,#44111);
#44064=APPLICATION_CONTEXT(
'Core Data for Automotive Mechanical Design Process');
#44065=PRODUCT_CONTEXT('part definition',#44064,'mechanical');
#44111=PRODUCT('Linear bushing housing','Linear bushing housing',
'Linear bushing housing',(#44065));
#44175=COLOUR_RGB('Dark Blue',0.08,0.2,0.34);
#44176=FILL_AREA_STYLE_COLOUR('',#44175);
#44177=FILL_AREA_STYLE('',(#44176));
#44178=SURFACE_STYLE_FILL_AREA(#44177);
#44179=SURFACE_SIDE_STYLE('',(#44178));
#44180=SURFACE_STYLE_USAGE(.BOTH.,#44179);
#44181=PRESENTATION_STYLE_ASSIGNMENT((#44180));
ENDSEC;
END-ISO-10303-21;
